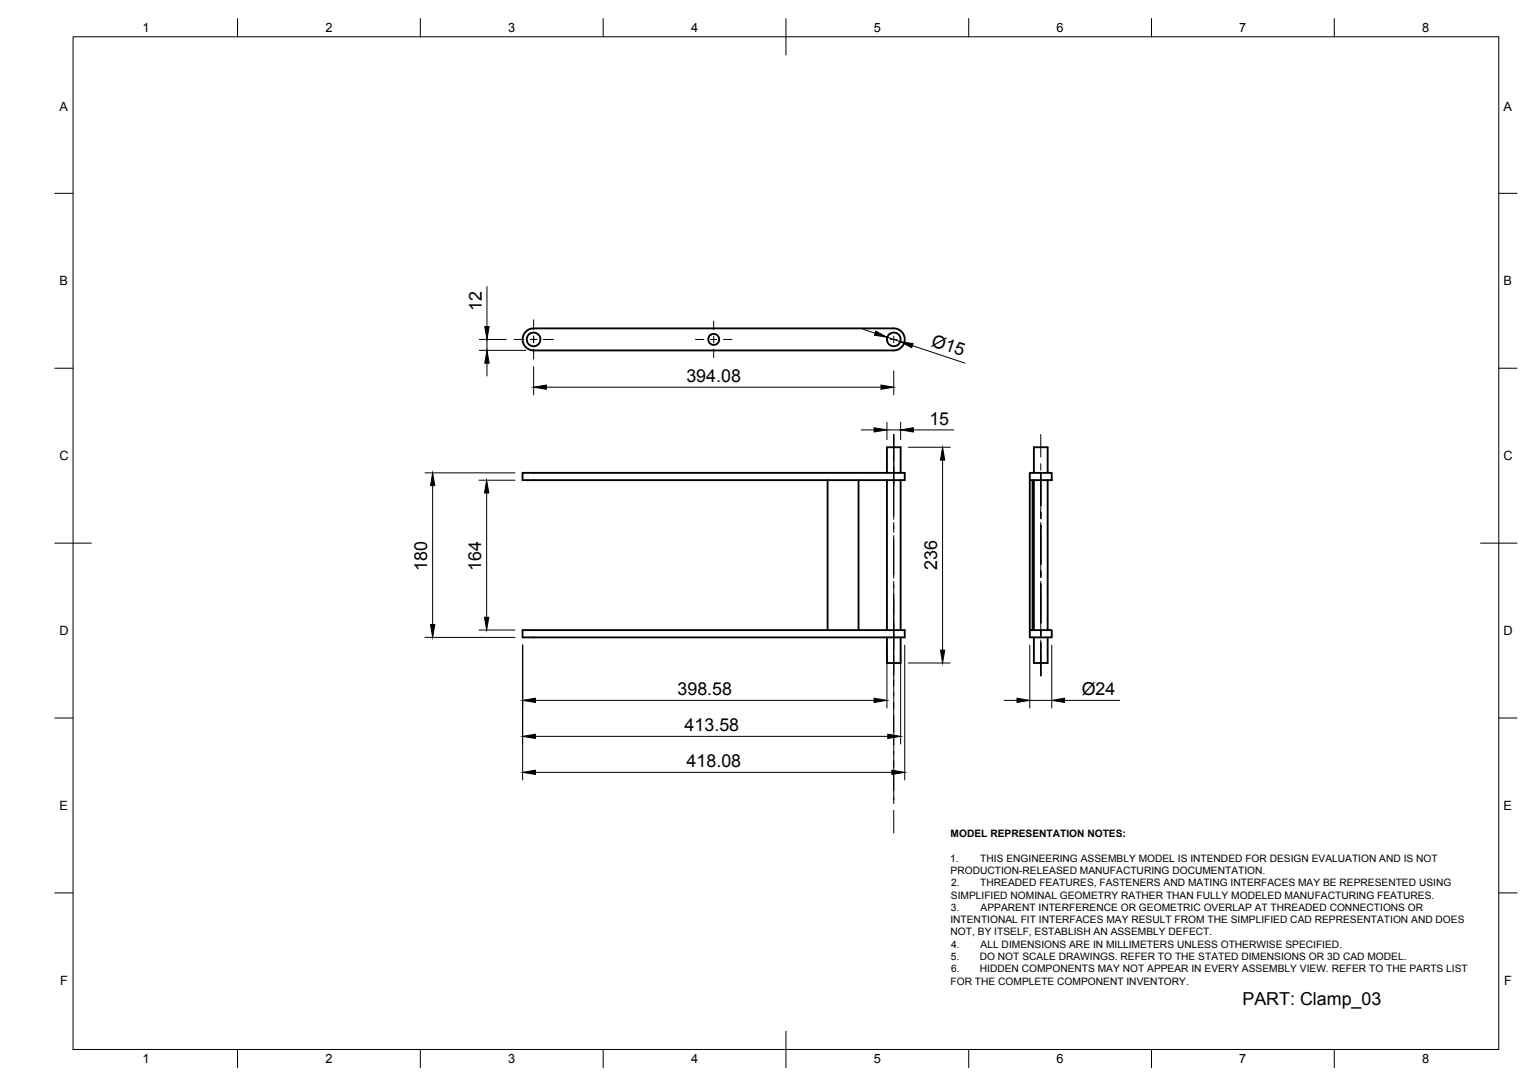
ISO-10303-21;
HEADER;
/* Generated by software containing ST-Developer
 * from STEP Tools, Inc. (www.steptools.com) 
 */

FILE_DESCRIPTION(
/* description */ (''),
/* implementation_level */ '2;1');

FILE_NAME(
/* name */ 'Clamp_03.step',
/* time_stamp */ '2026-10-05T15:35:09-07:00',
/* author */ (''),
/* organization */ (''),
/* preprocessor_version */ 'ST-DEVELOPER v20.2',
/* originating_system */ 'Autodesk Translation Framework v15.15.0.0',
/* authorisation */ '');

FILE_SCHEMA (('AUTOMOTIVE_DESIGN { 1 0 10303 214 3 1 1 }'));
ENDSEC;

DATA;
#10=MECHANICAL_DESIGN_GEOMETRIC_PRESENTATION_REPRESENTATION('',(#544),#74523);
#526=SHAPE_REPRESENTATION_RELATIONSHIP('SRR','None',#74559,#535);
#535=ADVANCED_BREP_SHAPE_REPRESENTATION('',(#553),#74515);
#544=STYLED_ITEM('',(#74612),#553);
#553=MANIFOLD_SOLID_BREP('Body1',#4723);
#569=FACE_BOUND('',#869,.T.);
#570=FACE_BOUND('',#870,.T.);
#571=FACE_BOUND('',#871,.T.);
#572=FACE_BOUND('',#873,.T.);
#573=FACE_BOUND('',#874,.T.);
#574=FACE_BOUND('',#875,.T.);
#575=FACE_BOUND('',#888,.T.);
#576=FACE_BOUND('',#889,.T.);
#577=FACE_BOUND('',#890,.T.);
#578=FACE_BOUND('',#892,.T.);
#579=FACE_BOUND('',#893,.T.);
#580=FACE_BOUND('',#894,.T.);
#623=PLANE('',#4902);
#624=PLANE('',#4906);
#625=PLANE('',#4907);
#626=PLANE('',#4911);
#627=PLANE('',#4912);
#628=PLANE('',#4913);
#629=PLANE('',#4914);
#630=PLANE('',#4915);
#631=PLANE('',#4919);
#632=PLANE('',#4923);
#633=PLANE('',#4927);
#634=PLANE('',#4928);
#708=FACE_OUTER_BOUND('',#860,.T.);
#709=FACE_OUTER_BOUND('',#861,.T.);
#710=FACE_OUTER_BOUND('',#862,.T.);
#711=FACE_OUTER_BOUND('',#863,.T.);
#712=FACE_OUTER_BOUND('',#864,.T.);
#713=FACE_OUTER_BOUND('',#865,.T.);
#714=FACE_OUTER_BOUND('',#866,.T.);
#715=FACE_OUTER_BOUND('',#867,.T.);
#716=FACE_OUTER_BOUND('',#868,.T.);
#717=FACE_OUTER_BOUND('',#872,.T.);
#718=FACE_OUTER_BOUND('',#876,.T.);
#719=FACE_OUTER_BOUND('',#877,.T.);
#720=FACE_OUTER_BOUND('',#878,.T.);
#721=FACE_OUTER_BOUND('',#879,.T.);
#722=FACE_OUTER_BOUND('',#880,.T.);
#723=FACE_OUTER_BOUND('',#881,.T.);
#724=FACE_OUTER_BOUND('',#882,.T.);
#725=FACE_OUTER_BOUND('',#883,.T.);
#726=FACE_OUTER_BOUND('',#884,.T.);
#727=FACE_OUTER_BOUND('',#885,.T.);
#728=FACE_OUTER_BOUND('',#886,.T.);
#729=FACE_OUTER_BOUND('',#887,.T.);
#730=FACE_OUTER_BOUND('',#891,.T.);
#860=EDGE_LOOP('',(#3102,#3103,#3104,#3105));
#861=EDGE_LOOP('',(#3106,#3107,#3108,#3109));
#862=EDGE_LOOP('',(#3110,#3111,#3112,#3113));
#863=EDGE_LOOP('',(#3114,#3115,#3116,#3117));
#864=EDGE_LOOP('',(#3118,#3119,#3120,#3121));
#865=EDGE_LOOP('',(#3122,#3123,#3124,#3125));
#866=EDGE_LOOP('',(#3126,#3127,#3128,#3129));
#867=EDGE_LOOP('',(#3130,#3131,#3132,#3133));
#868=EDGE_LOOP('',(#3134,#3135,#3136,#3137,#3138,#3139,#3140,#3141));
#869=EDGE_LOOP('',(#3142));
#870=EDGE_LOOP('',(#3143));
#871=EDGE_LOOP('',(#3144));
#872=EDGE_LOOP('',(#3145,#3146,#3147,#3148));
#873=EDGE_LOOP('',(#3149));
#874=EDGE_LOOP('',(#3150));
#875=EDGE_LOOP('',(#3151));
#876=EDGE_LOOP('',(#3152,#3153,#3154,#3155));
#877=EDGE_LOOP('',(#3156));
#878=EDGE_LOOP('',(#3157));
#879=EDGE_LOOP('',(#3158,#3159,#3160,#3161));
#880=EDGE_LOOP('',(#3162,#3163,#3164,#3165));
#881=EDGE_LOOP('',(#3166,#3167,#3168,#3169));
#882=EDGE_LOOP('',(#3170,#3171,#3172,#3173));
#883=EDGE_LOOP('',(#3174,#3175,#3176,#3177,#3178,#3179,#3180,#3181,#3182,
#3183,#3184,#3185));
#884=EDGE_LOOP('',(#3186,#3187,#3188,#3189));
#885=EDGE_LOOP('',(#3190,#3191,#3192,#3193));
#886=EDGE_LOOP('',(#3194,#3195,#3196,#3197));
#887=EDGE_LOOP('',(#3198,#3199,#3200,#3201,#3202,#3203,#3204,#3205));
#888=EDGE_LOOP('',(#3206));
#889=EDGE_LOOP('',(#3207));
#890=EDGE_LOOP('',(#3208));
#891=EDGE_LOOP('',(#3209,#3210,#3211,#3212));
#892=EDGE_LOOP('',(#3213));
#893=EDGE_LOOP('',(#3214));
#894=EDGE_LOOP('',(#3215));
#1066=LINE('',#5982,#1263);
#1067=LINE('',#5988,#1264);
#1068=LINE('',#5994,#1265);
#1069=LINE('',#6000,#1266);
#1070=LINE('',#6006,#1267);
#1071=LINE('',#6013,#1268);
#1072=LINE('',#6016,#1269);
#1073=LINE('',#6019,#1270);
#1074=LINE('',#6021,#1271);
#1075=LINE('',#6022,#1272);
#1076=LINE('',#6028,#1273);
#1077=LINE('',#6032,#1274);
#1078=LINE('',#6033,#1275);
#1079=LINE('',#6035,#1276);
#1080=LINE('',#6037,#1277);
#1081=LINE('',#6038,#1278);
#1082=LINE('',#6040,#1279);
#1083=LINE('',#6046,#1280);
#1084=LINE('',#6052,#1281);
#1085=LINE('',#6053,#1282);
#1086=LINE('',#6054,#1283);
#1087=LINE('',#6057,#1284);
#1088=LINE('',#6058,#1285);
#1089=LINE('',#6061,#1286);
#1090=LINE('',#6062,#1287);
#1091=LINE('',#6067,#1288);
#1092=LINE('',#6072,#1289);
#1093=LINE('',#6074,#1290);
#1094=LINE('',#6075,#1291);
#1095=LINE('',#6077,#1292);
#1096=LINE('',#6078,#1293);
#1097=LINE('',#6083,#1294);
#1098=LINE('',#6087,#1295);
#1099=LINE('',#6089,#1296);
#1100=LINE('',#6090,#1297);
#1263=VECTOR('',#5256,6.00000000000001);
#1264=VECTOR('',#5263,6.00000000000001);
#1265=VECTOR('',#5270,7.5);
#1266=VECTOR('',#5277,7.5);
#1267=VECTOR('',#5284,7.5);
#1268=VECTOR('',#5291,10.);
#1269=VECTOR('',#5294,10.);
#1270=VECTOR('',#5297,9.99999999999999);
#1271=VECTOR('',#5298,9.99999999999999);
#1272=VECTOR('',#5299,10.);
#1273=VECTOR('',#5306,10.);
#1274=VECTOR('',#5309,10.);
#1275=VECTOR('',#5310,9.99999999999999);
#1276=VECTOR('',#5311,9.99999999999999);
#1277=VECTOR('',#5312,10.);
#1278=VECTOR('',#5313,9.99999999999999);
#1279=VECTOR('',#5316,9.99999999999999);
#1280=VECTOR('',#5323,7.5);
#1281=VECTOR('',#5330,10.);
#1282=VECTOR('',#5331,10.);
#1283=VECTOR('',#5332,10.);
#1284=VECTOR('',#5335,9.99999999999999);
#1285=VECTOR('',#5336,10.);
#1286=VECTOR('',#5339,10.);
#1287=VECTOR('',#5340,10.);
#1288=VECTOR('',#5345,7.5);
#1289=VECTOR('',#5350,9.99999999999999);
#1290=VECTOR('',#5351,10.);
#1291=VECTOR('',#5352,9.99999999999999);
#1292=VECTOR('',#5353,9.99999999999999);
#1293=VECTOR('',#5354,10.);
#1294=VECTOR('',#5359,10.);
#1295=VECTOR('',#5364,9.99999999999999);
#1296=VECTOR('',#5365,10.);
#1297=VECTOR('',#5366,9.99999999999999);
#1436=CIRCLE('',#4885,6.00000000000001);
#1437=CIRCLE('',#4886,6.00000000000001);
#1438=CIRCLE('',#4888,6.00000000000001);
#1439=CIRCLE('',#4889,6.00000000000001);
#1440=CIRCLE('',#4891,7.5);
#1441=CIRCLE('',#4892,7.5);
#1442=CIRCLE('',#4894,7.5);
#1443=CIRCLE('',#4895,7.5);
#1444=CIRCLE('',#4897,7.5);
#1445=CIRCLE('',#4898,7.5);
#1446=CIRCLE('',#4900,12.);
#1447=CIRCLE('',#4901,12.);
#1448=CIRCLE('',#4904,12.);
#1449=CIRCLE('',#4905,12.);
#1450=CIRCLE('',#4908,7.5);
#1451=CIRCLE('',#4910,7.5);
#1452=CIRCLE('',#4917,7.5);
#1453=CIRCLE('',#4918,7.5);
#1454=CIRCLE('',#4921,12.);
#1455=CIRCLE('',#4922,12.);
#1456=CIRCLE('',#4925,12.);
#1457=CIRCLE('',#4926,12.);
#1570=VERTEX_POINT('',#5979);
#1571=VERTEX_POINT('',#5981);
#1572=VERTEX_POINT('',#5985);
#1573=VERTEX_POINT('',#5987);
#1574=VERTEX_POINT('',#5991);
#1575=VERTEX_POINT('',#5993);
#1576=VERTEX_POINT('',#5997);
#1577=VERTEX_POINT('',#5999);
#1578=VERTEX_POINT('',#6003);
#1579=VERTEX_POINT('',#6005);
#1580=VERTEX_POINT('',#6009);
#1581=VERTEX_POINT('',#6010);
#1582=VERTEX_POINT('',#6012);
#1583=VERTEX_POINT('',#6014);
#1584=VERTEX_POINT('',#6018);
#1585=VERTEX_POINT('',#6020);
#1586=VERTEX_POINT('',#6024);
#1587=VERTEX_POINT('',#6026);
#1588=VERTEX_POINT('',#6030);
#1589=VERTEX_POINT('',#6031);
#1590=VERTEX_POINT('',#6034);
#1591=VERTEX_POINT('',#6036);
#1592=VERTEX_POINT('',#6041);
#1593=VERTEX_POINT('',#6044);
#1594=VERTEX_POINT('',#6050);
#1595=VERTEX_POINT('',#6051);
#1596=VERTEX_POINT('',#6056);
#1597=VERTEX_POINT('',#6060);
#1598=VERTEX_POINT('',#6064);
#1599=VERTEX_POINT('',#6066);
#1600=VERTEX_POINT('',#6070);
#1601=VERTEX_POINT('',#6071);
#1602=VERTEX_POINT('',#6073);
#1603=VERTEX_POINT('',#6076);
#1604=VERTEX_POINT('',#6080);
#1605=VERTEX_POINT('',#6082);
#1606=VERTEX_POINT('',#6086);
#1607=VERTEX_POINT('',#6088);
#2252=EDGE_CURVE('',#1570,#1570,#1436,.T.);
#2253=EDGE_CURVE('',#1570,#1571,#1066,.T.);
#2254=EDGE_CURVE('',#1571,#1571,#1437,.T.);
#2255=EDGE_CURVE('',#1572,#1572,#1438,.T.);
#2256=EDGE_CURVE('',#1572,#1573,#1067,.T.);
#2257=EDGE_CURVE('',#1573,#1573,#1439,.T.);
#2258=EDGE_CURVE('',#1574,#1574,#1440,.T.);
#2259=EDGE_CURVE('',#1574,#1575,#1068,.T.);
#2260=EDGE_CURVE('',#1575,#1575,#1441,.T.);
#2261=EDGE_CURVE('',#1576,#1576,#1442,.T.);
#2262=EDGE_CURVE('',#1576,#1577,#1069,.T.);
#2263=EDGE_CURVE('',#1577,#1577,#1443,.T.);
#2264=EDGE_CURVE('',#1578,#1578,#1444,.T.);
#2265=EDGE_CURVE('',#1578,#1579,#1070,.T.);
#2266=EDGE_CURVE('',#1579,#1579,#1445,.T.);
#2267=EDGE_CURVE('',#1580,#1581,#1446,.T.);
#2268=EDGE_CURVE('',#1581,#1582,#1071,.T.);
#2269=EDGE_CURVE('',#1583,#1582,#1447,.T.);
#2270=EDGE_CURVE('',#1580,#1583,#1072,.T.);
#2271=EDGE_CURVE('',#1584,#1580,#1073,.T.);
#2272=EDGE_CURVE('',#1585,#1583,#1074,.T.);
#2273=EDGE_CURVE('',#1584,#1585,#1075,.T.);
#2274=EDGE_CURVE('',#1586,#1584,#1448,.T.);
#2275=EDGE_CURVE('',#1587,#1585,#1449,.T.);
#2276=EDGE_CURVE('',#1586,#1587,#1076,.T.);
#2277=EDGE_CURVE('',#1588,#1589,#1077,.T.);
#2278=EDGE_CURVE('',#1589,#1587,#1078,.T.);
#2279=EDGE_CURVE('',#1582,#1590,#1079,.T.);
#2280=EDGE_CURVE('',#1590,#1591,#1080,.T.);
#2281=EDGE_CURVE('',#1591,#1588,#1081,.T.);
#2282=EDGE_CURVE('',#1581,#1586,#1082,.T.);
#2283=EDGE_CURVE('',#1592,#1592,#1450,.T.);
#2284=EDGE_CURVE('',#1593,#1593,#1451,.T.);
#2285=EDGE_CURVE('',#1593,#1592,#1083,.T.);
#2286=EDGE_CURVE('',#1594,#1595,#1084,.T.);
#2287=EDGE_CURVE('',#1594,#1589,#1085,.T.);
#2288=EDGE_CURVE('',#1595,#1588,#1086,.T.);
#2289=EDGE_CURVE('',#1595,#1596,#1087,.T.);
#2290=EDGE_CURVE('',#1596,#1591,#1088,.T.);
#2291=EDGE_CURVE('',#1596,#1597,#1089,.T.);
#2292=EDGE_CURVE('',#1597,#1590,#1090,.T.);
#2293=EDGE_CURVE('',#1598,#1598,#1452,.T.);
#2294=EDGE_CURVE('',#1598,#1599,#1091,.T.);
#2295=EDGE_CURVE('',#1599,#1599,#1453,.T.);
#2296=EDGE_CURVE('',#1600,#1601,#1092,.T.);
#2297=EDGE_CURVE('',#1600,#1602,#1093,.T.);
#2298=EDGE_CURVE('',#1602,#1597,#1094,.T.);
#2299=EDGE_CURVE('',#1594,#1603,#1095,.T.);
#2300=EDGE_CURVE('',#1601,#1603,#1096,.T.);
#2301=EDGE_CURVE('',#1604,#1600,#1454,.T.);
#2302=EDGE_CURVE('',#1604,#1605,#1097,.T.);
#2303=EDGE_CURVE('',#1605,#1602,#1455,.T.);
#2304=EDGE_CURVE('',#1606,#1604,#1098,.T.);
#2305=EDGE_CURVE('',#1606,#1607,#1099,.T.);
#2306=EDGE_CURVE('',#1607,#1605,#1100,.T.);
#2307=EDGE_CURVE('',#1601,#1606,#1456,.T.);
#2308=EDGE_CURVE('',#1603,#1607,#1457,.T.);
#3102=ORIENTED_EDGE('',*,*,#2252,.F.);
#3103=ORIENTED_EDGE('',*,*,#2253,.T.);
#3104=ORIENTED_EDGE('',*,*,#2254,.F.);
#3105=ORIENTED_EDGE('',*,*,#2253,.F.);
#3106=ORIENTED_EDGE('',*,*,#2255,.F.);
#3107=ORIENTED_EDGE('',*,*,#2256,.T.);
#3108=ORIENTED_EDGE('',*,*,#2257,.F.);
#3109=ORIENTED_EDGE('',*,*,#2256,.F.);
#3110=ORIENTED_EDGE('',*,*,#2258,.F.);
#3111=ORIENTED_EDGE('',*,*,#2259,.T.);
#3112=ORIENTED_EDGE('',*,*,#2260,.T.);
#3113=ORIENTED_EDGE('',*,*,#2259,.F.);
#3114=ORIENTED_EDGE('',*,*,#2261,.T.);
#3115=ORIENTED_EDGE('',*,*,#2262,.T.);
#3116=ORIENTED_EDGE('',*,*,#2263,.T.);
#3117=ORIENTED_EDGE('',*,*,#2262,.F.);
#3118=ORIENTED_EDGE('',*,*,#2264,.T.);
#3119=ORIENTED_EDGE('',*,*,#2265,.T.);
#3120=ORIENTED_EDGE('',*,*,#2266,.F.);
#3121=ORIENTED_EDGE('',*,*,#2265,.F.);
#3122=ORIENTED_EDGE('',*,*,#2267,.T.);
#3123=ORIENTED_EDGE('',*,*,#2268,.T.);
#3124=ORIENTED_EDGE('',*,*,#2269,.F.);
#3125=ORIENTED_EDGE('',*,*,#2270,.F.);
#3126=ORIENTED_EDGE('',*,*,#2271,.T.);
#3127=ORIENTED_EDGE('',*,*,#2270,.T.);
#3128=ORIENTED_EDGE('',*,*,#2272,.F.);
#3129=ORIENTED_EDGE('',*,*,#2273,.F.);
#3130=ORIENTED_EDGE('',*,*,#2274,.T.);
#3131=ORIENTED_EDGE('',*,*,#2273,.T.);
#3132=ORIENTED_EDGE('',*,*,#2275,.F.);
#3133=ORIENTED_EDGE('',*,*,#2276,.F.);
#3134=ORIENTED_EDGE('',*,*,#2277,.T.);
#3135=ORIENTED_EDGE('',*,*,#2278,.T.);
#3136=ORIENTED_EDGE('',*,*,#2275,.T.);
#3137=ORIENTED_EDGE('',*,*,#2272,.T.);
#3138=ORIENTED_EDGE('',*,*,#2269,.T.);
#3139=ORIENTED_EDGE('',*,*,#2279,.T.);
#3140=ORIENTED_EDGE('',*,*,#2280,.T.);
#3141=ORIENTED_EDGE('',*,*,#2281,.T.);
#3142=ORIENTED_EDGE('',*,*,#2252,.T.);
#3143=ORIENTED_EDGE('',*,*,#2261,.F.);
#3144=ORIENTED_EDGE('',*,*,#2266,.T.);
#3145=ORIENTED_EDGE('',*,*,#2274,.F.);
#3146=ORIENTED_EDGE('',*,*,#2282,.F.);
#3147=ORIENTED_EDGE('',*,*,#2267,.F.);
#3148=ORIENTED_EDGE('',*,*,#2271,.F.);
#3149=ORIENTED_EDGE('',*,*,#2254,.T.);
#3150=ORIENTED_EDGE('',*,*,#2283,.F.);
#3151=ORIENTED_EDGE('',*,*,#2264,.F.);
#3152=ORIENTED_EDGE('',*,*,#2284,.T.);
#3153=ORIENTED_EDGE('',*,*,#2285,.T.);
#3154=ORIENTED_EDGE('',*,*,#2283,.T.);
#3155=ORIENTED_EDGE('',*,*,#2285,.F.);
#3156=ORIENTED_EDGE('',*,*,#2284,.F.);
#3157=ORIENTED_EDGE('',*,*,#2260,.F.);
#3158=ORIENTED_EDGE('',*,*,#2286,.F.);
#3159=ORIENTED_EDGE('',*,*,#2287,.T.);
#3160=ORIENTED_EDGE('',*,*,#2277,.F.);
#3161=ORIENTED_EDGE('',*,*,#2288,.F.);
#3162=ORIENTED_EDGE('',*,*,#2289,.F.);
#3163=ORIENTED_EDGE('',*,*,#2288,.T.);
#3164=ORIENTED_EDGE('',*,*,#2281,.F.);
#3165=ORIENTED_EDGE('',*,*,#2290,.F.);
#3166=ORIENTED_EDGE('',*,*,#2291,.F.);
#3167=ORIENTED_EDGE('',*,*,#2290,.T.);
#3168=ORIENTED_EDGE('',*,*,#2280,.F.);
#3169=ORIENTED_EDGE('',*,*,#2292,.F.);
#3170=ORIENTED_EDGE('',*,*,#2293,.T.);
#3171=ORIENTED_EDGE('',*,*,#2294,.T.);
#3172=ORIENTED_EDGE('',*,*,#2295,.F.);
#3173=ORIENTED_EDGE('',*,*,#2294,.F.);
#3174=ORIENTED_EDGE('',*,*,#2296,.F.);
#3175=ORIENTED_EDGE('',*,*,#2297,.T.);
#3176=ORIENTED_EDGE('',*,*,#2298,.T.);
#3177=ORIENTED_EDGE('',*,*,#2292,.T.);
#3178=ORIENTED_EDGE('',*,*,#2279,.F.);
#3179=ORIENTED_EDGE('',*,*,#2268,.F.);
#3180=ORIENTED_EDGE('',*,*,#2282,.T.);
#3181=ORIENTED_EDGE('',*,*,#2276,.T.);
#3182=ORIENTED_EDGE('',*,*,#2278,.F.);
#3183=ORIENTED_EDGE('',*,*,#2287,.F.);
#3184=ORIENTED_EDGE('',*,*,#2299,.T.);
#3185=ORIENTED_EDGE('',*,*,#2300,.F.);
#3186=ORIENTED_EDGE('',*,*,#2301,.F.);
#3187=ORIENTED_EDGE('',*,*,#2302,.T.);
#3188=ORIENTED_EDGE('',*,*,#2303,.T.);
#3189=ORIENTED_EDGE('',*,*,#2297,.F.);
#3190=ORIENTED_EDGE('',*,*,#2304,.F.);
#3191=ORIENTED_EDGE('',*,*,#2305,.T.);
#3192=ORIENTED_EDGE('',*,*,#2306,.T.);
#3193=ORIENTED_EDGE('',*,*,#2302,.F.);
#3194=ORIENTED_EDGE('',*,*,#2307,.F.);
#3195=ORIENTED_EDGE('',*,*,#2300,.T.);
#3196=ORIENTED_EDGE('',*,*,#2308,.T.);
#3197=ORIENTED_EDGE('',*,*,#2305,.F.);
#3198=ORIENTED_EDGE('',*,*,#2291,.T.);
#3199=ORIENTED_EDGE('',*,*,#2298,.F.);
#3200=ORIENTED_EDGE('',*,*,#2303,.F.);
#3201=ORIENTED_EDGE('',*,*,#2306,.F.);
#3202=ORIENTED_EDGE('',*,*,#2308,.F.);
#3203=ORIENTED_EDGE('',*,*,#2299,.F.);
#3204=ORIENTED_EDGE('',*,*,#2286,.T.);
#3205=ORIENTED_EDGE('',*,*,#2289,.T.);
#3206=ORIENTED_EDGE('',*,*,#2255,.T.);
#3207=ORIENTED_EDGE('',*,*,#2263,.F.);
#3208=ORIENTED_EDGE('',*,*,#2293,.F.);
#3209=ORIENTED_EDGE('',*,*,#2307,.T.);
#3210=ORIENTED_EDGE('',*,*,#2304,.T.);
#3211=ORIENTED_EDGE('',*,*,#2301,.T.);
#3212=ORIENTED_EDGE('',*,*,#2296,.T.);
#3213=ORIENTED_EDGE('',*,*,#2257,.T.);
#3214=ORIENTED_EDGE('',*,*,#2258,.T.);
#3215=ORIENTED_EDGE('',*,*,#2295,.T.);
#4526=CYLINDRICAL_SURFACE('',#4884,6.00000000000001);
#4527=CYLINDRICAL_SURFACE('',#4887,6.00000000000001);
#4528=CYLINDRICAL_SURFACE('',#4890,7.5);
#4529=CYLINDRICAL_SURFACE('',#4893,7.5);
#4530=CYLINDRICAL_SURFACE('',#4896,7.5);
#4531=CYLINDRICAL_SURFACE('',#4899,12.);
#4532=CYLINDRICAL_SURFACE('',#4903,12.);
#4533=CYLINDRICAL_SURFACE('',#4909,7.5);
#4534=CYLINDRICAL_SURFACE('',#4916,7.5);
#4535=CYLINDRICAL_SURFACE('',#4920,12.);
#4536=CYLINDRICAL_SURFACE('',#4924,12.);
#4604=ADVANCED_FACE('',(#708),#4526,.F.);
#4605=ADVANCED_FACE('',(#709),#4527,.F.);
#4606=ADVANCED_FACE('',(#710),#4528,.T.);
#4607=ADVANCED_FACE('',(#711),#4529,.T.);
#4608=ADVANCED_FACE('',(#712),#4530,.F.);
#4609=ADVANCED_FACE('',(#713),#4531,.T.);
#4610=ADVANCED_FACE('',(#714),#623,.T.);
#4611=ADVANCED_FACE('',(#715),#4532,.T.);
#4612=ADVANCED_FACE('',(#716,#569,#570,#571),#624,.T.);
#4613=ADVANCED_FACE('',(#717,#572,#573,#574),#625,.F.);
#4614=ADVANCED_FACE('',(#718),#4533,.T.);
#4615=ADVANCED_FACE('',(#719),#626,.T.);
#4616=ADVANCED_FACE('',(#720),#627,.F.);
#4617=ADVANCED_FACE('',(#721),#628,.T.);
#4618=ADVANCED_FACE('',(#722),#629,.T.);
#4619=ADVANCED_FACE('',(#723),#630,.T.);
#4620=ADVANCED_FACE('',(#724),#4534,.F.);
#4621=ADVANCED_FACE('',(#725),#631,.F.);
#4622=ADVANCED_FACE('',(#726),#4535,.T.);
#4623=ADVANCED_FACE('',(#727),#632,.F.);
#4624=ADVANCED_FACE('',(#728),#4536,.T.);
#4625=ADVANCED_FACE('',(#729,#575,#576,#577),#633,.F.);
#4626=ADVANCED_FACE('',(#730,#578,#579,#580),#634,.T.);
#4723=CLOSED_SHELL('',(#4604,#4605,#4606,#4607,#4608,#4609,#4610,#4611,
#4612,#4613,#4614,#4615,#4616,#4617,#4618,#4619,#4620,#4621,#4622,#4623,
#4624,#4625,#4626));
#4883=AXIS2_PLACEMENT_3D('',#5977,#5250,#5251);
#4884=AXIS2_PLACEMENT_3D('',#5978,#5252,#5253);
#4885=AXIS2_PLACEMENT_3D('',#5980,#5254,#5255);
#4886=AXIS2_PLACEMENT_3D('',#5983,#5257,#5258);
#4887=AXIS2_PLACEMENT_3D('',#5984,#5259,#5260);
#4888=AXIS2_PLACEMENT_3D('',#5986,#5261,#5262);
#4889=AXIS2_PLACEMENT_3D('',#5989,#5264,#5265);
#4890=AXIS2_PLACEMENT_3D('',#5990,#5266,#5267);
#4891=AXIS2_PLACEMENT_3D('',#5992,#5268,#5269);
#4892=AXIS2_PLACEMENT_3D('',#5995,#5271,#5272);
#4893=AXIS2_PLACEMENT_3D('',#5996,#5273,#5274);
#4894=AXIS2_PLACEMENT_3D('',#5998,#5275,#5276);
#4895=AXIS2_PLACEMENT_3D('',#6001,#5278,#5279);
#4896=AXIS2_PLACEMENT_3D('',#6002,#5280,#5281);
#4897=AXIS2_PLACEMENT_3D('',#6004,#5282,#5283);
#4898=AXIS2_PLACEMENT_3D('',#6007,#5285,#5286);
#4899=AXIS2_PLACEMENT_3D('',#6008,#5287,#5288);
#4900=AXIS2_PLACEMENT_3D('',#6011,#5289,#5290);
#4901=AXIS2_PLACEMENT_3D('',#6015,#5292,#5293);
#4902=AXIS2_PLACEMENT_3D('',#6017,#5295,#5296);
#4903=AXIS2_PLACEMENT_3D('',#6023,#5300,#5301);
#4904=AXIS2_PLACEMENT_3D('',#6025,#5302,#5303);
#4905=AXIS2_PLACEMENT_3D('',#6027,#5304,#5305);
#4906=AXIS2_PLACEMENT_3D('',#6029,#5307,#5308);
#4907=AXIS2_PLACEMENT_3D('',#6039,#5314,#5315);
#4908=AXIS2_PLACEMENT_3D('',#6042,#5317,#5318);
#4909=AXIS2_PLACEMENT_3D('',#6043,#5319,#5320);
#4910=AXIS2_PLACEMENT_3D('',#6045,#5321,#5322);
#4911=AXIS2_PLACEMENT_3D('',#6047,#5324,#5325);
#4912=AXIS2_PLACEMENT_3D('',#6048,#5326,#5327);
#4913=AXIS2_PLACEMENT_3D('',#6049,#5328,#5329);
#4914=AXIS2_PLACEMENT_3D('',#6055,#5333,#5334);
#4915=AXIS2_PLACEMENT_3D('',#6059,#5337,#5338);
#4916=AXIS2_PLACEMENT_3D('',#6063,#5341,#5342);
#4917=AXIS2_PLACEMENT_3D('',#6065,#5343,#5344);
#4918=AXIS2_PLACEMENT_3D('',#6068,#5346,#5347);
#4919=AXIS2_PLACEMENT_3D('',#6069,#5348,#5349);
#4920=AXIS2_PLACEMENT_3D('',#6079,#5355,#5356);
#4921=AXIS2_PLACEMENT_3D('',#6081,#5357,#5358);
#4922=AXIS2_PLACEMENT_3D('',#6084,#5360,#5361);
#4923=AXIS2_PLACEMENT_3D('',#6085,#5362,#5363);
#4924=AXIS2_PLACEMENT_3D('',#6091,#5367,#5368);
#4925=AXIS2_PLACEMENT_3D('',#6092,#5369,#5370);
#4926=AXIS2_PLACEMENT_3D('',#6093,#5371,#5372);
#4927=AXIS2_PLACEMENT_3D('',#6094,#5373,#5374);
#4928=AXIS2_PLACEMENT_3D('',#6095,#5375,#5376);
#5250=DIRECTION('axis',(0.,0.,1.));
#5251=DIRECTION('refdir',(1.,0.,0.));
#5252=DIRECTION('center_axis',(0.,-1.,0.));
#5253=DIRECTION('ref_axis',(1.,0.,0.));
#5254=DIRECTION('center_axis',(0.,-1.,0.));
#5255=DIRECTION('ref_axis',(1.,0.,0.));
#5256=DIRECTION('',(0.,-1.,0.));
#5257=DIRECTION('center_axis',(0.,1.,0.));
#5258=DIRECTION('ref_axis',(1.,0.,0.));
#5259=DIRECTION('center_axis',(0.,1.,0.));
#5260=DIRECTION('ref_axis',(1.,0.,0.));
#5261=DIRECTION('center_axis',(0.,1.,0.));
#5262=DIRECTION('ref_axis',(1.,0.,0.));
#5263=DIRECTION('',(0.,1.,0.));
#5264=DIRECTION('center_axis',(0.,-1.,0.));
#5265=DIRECTION('ref_axis',(1.,0.,0.));
#5266=DIRECTION('center_axis',(-3.66477378287572E-33,-1.,2.99251489117293E-17));
#5267=DIRECTION('ref_axis',(1.,3.66477378287573E-33,2.44929359829471E-16));
#5268=DIRECTION('center_axis',(0.,-1.,0.));
#5269=DIRECTION('ref_axis',(1.,0.,0.));
#5270=DIRECTION('',(3.66477378287572E-33,1.,-2.99251489117293E-17));
#5271=DIRECTION('center_axis',(-3.66477378287572E-33,-1.,2.99251489117293E-17));
#5272=DIRECTION('ref_axis',(1.,3.66477378287573E-33,2.44929359829471E-16));
#5273=DIRECTION('center_axis',(-3.66477378287572E-33,-1.,2.99251489117293E-17));
#5274=DIRECTION('ref_axis',(1.,3.66477378287573E-33,2.44929359829471E-16));
#5275=DIRECTION('center_axis',(0.,1.,0.));
#5276=DIRECTION('ref_axis',(1.,0.,2.44929359829471E-16));
#5277=DIRECTION('',(3.66477378287572E-33,1.,-2.99251489117293E-17));
#5278=DIRECTION('center_axis',(0.,-1.,0.));
#5279=DIRECTION('ref_axis',(1.,0.,0.));
#5280=DIRECTION('center_axis',(0.,1.,0.));
#5281=DIRECTION('ref_axis',(1.,0.,0.));
#5282=DIRECTION('center_axis',(0.,-1.,0.));
#5283=DIRECTION('ref_axis',(1.,0.,0.));
#5284=DIRECTION('',(0.,1.,0.));
#5285=DIRECTION('center_axis',(0.,-1.,0.));
#5286=DIRECTION('ref_axis',(1.,0.,0.));
#5287=DIRECTION('center_axis',(0.,1.,0.));
#5288=DIRECTION('ref_axis',(0.812015371342714,0.,0.583636048152574));
#5289=DIRECTION('center_axis',(0.,1.,0.));
#5290=DIRECTION('ref_axis',(0.812015371342714,0.,0.583636048152574));
#5291=DIRECTION('',(0.,1.,0.));
#5292=DIRECTION('center_axis',(0.,1.,0.));
#5293=DIRECTION('ref_axis',(0.812015371342714,0.,0.583636048152574));
#5294=DIRECTION('',(0.,1.,0.));
#5295=DIRECTION('center_axis',(0.812015371342714,0.,0.583636048152575));
#5296=DIRECTION('ref_axis',(0.583636048152575,0.,-0.812015371342714));
#5297=DIRECTION('',(0.583636048152575,0.,-0.812015371342714));
#5298=DIRECTION('',(0.583636048152575,0.,-0.812015371342714));
#5299=DIRECTION('',(0.,1.,0.));
#5300=DIRECTION('center_axis',(0.,1.,0.));
#5301=DIRECTION('ref_axis',(-0.812015371342714,0.,-0.583636048152575));
#5302=DIRECTION('center_axis',(0.,1.,0.));
#5303=DIRECTION('ref_axis',(-0.812015371342714,0.,-0.583636048152575));
#5304=DIRECTION('center_axis',(0.,1.,0.));
#5305=DIRECTION('ref_axis',(-0.812015371342714,0.,-0.583636048152575));
#5306=DIRECTION('',(0.,1.,0.));
#5307=DIRECTION('center_axis',(0.,1.,0.));
#5308=DIRECTION('ref_axis',(1.,0.,0.));
#5309=DIRECTION('',(-0.812015371342711,0.,-0.583636048152579));
#5310=DIRECTION('',(-0.583636048152575,0.,0.812015371342714));
#5311=DIRECTION('',(-0.583636048152575,0.,0.812015371342714));
#5312=DIRECTION('',(0.812015371342709,0.,0.583636048152581));
#5313=DIRECTION('',(-0.583636048152575,0.,0.812015371342714));
#5314=DIRECTION('center_axis',(0.,1.,0.));
#5315=DIRECTION('ref_axis',(1.,0.,0.));
#5316=DIRECTION('',(-0.583636048152575,0.,0.812015371342714));
#5317=DIRECTION('center_axis',(0.,-1.,0.));
#5318=DIRECTION('ref_axis',(1.,0.,2.44929359829471E-16));
#5319=DIRECTION('center_axis',(-3.66477378287572E-33,-1.,2.99251489117293E-17));
#5320=DIRECTION('ref_axis',(1.,3.66477378287573E-33,2.44929359829471E-16));
#5321=DIRECTION('center_axis',(3.66477378287572E-33,1.,-2.99251489117293E-17));
#5322=DIRECTION('ref_axis',(1.,3.66477378287573E-33,2.44929359829471E-16));
#5323=DIRECTION('',(3.66477378287572E-33,1.,-2.99251489117293E-17));
#5324=DIRECTION('center_axis',(-3.66477378287572E-33,-1.,2.99251489117293E-17));
#5325=DIRECTION('ref_axis',(1.,3.66477378287573E-33,2.44929359829471E-16));
#5326=DIRECTION('center_axis',(-3.66477378287572E-33,-1.,2.99251489117293E-17));
#5327=DIRECTION('ref_axis',(1.,3.66477378287573E-33,2.44929359829471E-16));
#5328=DIRECTION('center_axis',(-0.583636048152579,0.,0.812015371342711));
#5329=DIRECTION('ref_axis',(-0.812015371342711,0.,-0.583636048152579));
#5330=DIRECTION('',(0.812015371342711,0.,0.583636048152579));
#5331=DIRECTION('',(0.,-1.,0.));
#5332=DIRECTION('',(0.,-1.,0.));
#5333=DIRECTION('center_axis',(0.812015371342714,0.,0.583636048152575));
#5334=DIRECTION('ref_axis',(-0.583636048152575,0.,0.812015371342714));
#5335=DIRECTION('',(0.583636048152575,0.,-0.812015371342714));
#5336=DIRECTION('',(0.,-1.,0.));
#5337=DIRECTION('center_axis',(0.583636048152581,0.,-0.812015371342709));
#5338=DIRECTION('ref_axis',(0.812015371342709,0.,0.583636048152581));
#5339=DIRECTION('',(-0.812015371342709,0.,-0.583636048152581));
#5340=DIRECTION('',(0.,-1.,0.));
#5341=DIRECTION('center_axis',(0.,1.,0.));
#5342=DIRECTION('ref_axis',(1.,0.,0.));
#5343=DIRECTION('center_axis',(0.,-1.,0.));
#5344=DIRECTION('ref_axis',(1.,0.,0.));
#5345=DIRECTION('',(0.,1.,0.));
#5346=DIRECTION('center_axis',(0.,-1.,0.));
#5347=DIRECTION('ref_axis',(1.,0.,0.));
#5348=DIRECTION('center_axis',(0.812015371342714,0.,0.583636048152575));
#5349=DIRECTION('ref_axis',(-0.583636048152575,0.,0.812015371342714));
#5350=DIRECTION('',(-0.583636048152575,0.,0.812015371342714));
#5351=DIRECTION('',(0.,-1.,0.));
#5352=DIRECTION('',(-0.583636048152575,0.,0.812015371342714));
#5353=DIRECTION('',(-0.583636048152575,0.,0.812015371342714));
#5354=DIRECTION('',(0.,-1.,0.));
#5355=DIRECTION('center_axis',(0.,1.,0.));
#5356=DIRECTION('ref_axis',(0.812015371342714,0.,0.583636048152574));
#5357=DIRECTION('center_axis',(0.,1.,0.));
#5358=DIRECTION('ref_axis',(0.812015371342714,0.,0.583636048152574));
#5359=DIRECTION('',(0.,-1.,0.));
#5360=DIRECTION('center_axis',(0.,1.,0.));
#5361=DIRECTION('ref_axis',(0.812015371342714,0.,0.583636048152574));
#5362=DIRECTION('center_axis',(-0.812015371342714,0.,-0.583636048152575));
#5363=DIRECTION('ref_axis',(0.583636048152575,0.,-0.812015371342714));
#5364=DIRECTION('',(0.583636048152575,0.,-0.812015371342714));
#5365=DIRECTION('',(0.,-1.,0.));
#5366=DIRECTION('',(0.583636048152575,0.,-0.812015371342714));
#5367=DIRECTION('center_axis',(0.,1.,0.));
#5368=DIRECTION('ref_axis',(-0.812015371342714,0.,-0.583636048152575));
#5369=DIRECTION('center_axis',(0.,1.,0.));
#5370=DIRECTION('ref_axis',(-0.812015371342714,0.,-0.583636048152575));
#5371=DIRECTION('center_axis',(0.,1.,0.));
#5372=DIRECTION('ref_axis',(-0.812015371342714,0.,-0.583636048152575));
#5373=DIRECTION('center_axis',(0.,1.,0.));
#5374=DIRECTION('ref_axis',(1.,0.,0.));
#5375=DIRECTION('center_axis',(0.,1.,0.));
#5376=DIRECTION('ref_axis',(1.,0.,0.));
#5977=CARTESIAN_POINT('',(0.,0.,0.));
#5978=CARTESIAN_POINT('Origin',(60.231676812499,-90.,175.));
#5979=CARTESIAN_POINT('',(54.231676812499,-82.,175.));
#5980=CARTESIAN_POINT('Origin',(60.231676812499,-82.,175.));
#5981=CARTESIAN_POINT('',(54.231676812499,-90.,175.));
#5982=CARTESIAN_POINT('',(54.231676812499,-90.,175.));
#5983=CARTESIAN_POINT('Origin',(60.231676812499,-90.,175.));
#5984=CARTESIAN_POINT('Origin',(60.231676812499,-90.,175.));
#5985=CARTESIAN_POINT('',(54.231676812499,82.,175.));
#5986=CARTESIAN_POINT('Origin',(60.231676812499,82.,175.));
#5987=CARTESIAN_POINT('',(54.231676812499,90.,175.));
#5988=CARTESIAN_POINT('',(54.231676812499,-90.,175.));
#5989=CARTESIAN_POINT('Origin',(60.231676812499,90.,175.));
#5990=CARTESIAN_POINT('Origin',(-54.768323187501,4.78802382587669E-15,335.));
#5991=CARTESIAN_POINT('',(-62.268323187501,90.,335.));
#5992=CARTESIAN_POINT('Origin',(-54.768323187501,90.,335.));
#5993=CARTESIAN_POINT('',(-62.268323187501,118.,335.));
#5994=CARTESIAN_POINT('',(-62.268323187501,4.78802382587669E-15,335.));
#5995=CARTESIAN_POINT('Origin',(-54.768323187501,118.,335.));
#5996=CARTESIAN_POINT('Origin',(-54.768323187501,4.78802382587669E-15,335.));
#5997=CARTESIAN_POINT('',(-62.268323187501,-82.,335.));
#5998=CARTESIAN_POINT('Origin',(-54.768323187501,-82.,335.));
#5999=CARTESIAN_POINT('',(-62.268323187501,82.,335.));
#6000=CARTESIAN_POINT('',(-62.268323187501,4.78802382587669E-15,335.));
#6001=CARTESIAN_POINT('Origin',(-54.768323187501,82.,335.));
#6002=CARTESIAN_POINT('Origin',(175.231676812499,-90.,15.));
#6003=CARTESIAN_POINT('',(167.731676812499,-90.,15.));
#6004=CARTESIAN_POINT('Origin',(175.231676812499,-90.,15.));
#6005=CARTESIAN_POINT('',(167.731676812499,-82.,15.));
#6006=CARTESIAN_POINT('',(167.731676812499,-90.,15.));
#6007=CARTESIAN_POINT('Origin',(175.231676812499,-82.,15.));
#6008=CARTESIAN_POINT('Origin',(175.231676812499,-90.,15.));
#6009=CARTESIAN_POINT('',(184.975861268612,-90.,22.0036325778309));
#6010=CARTESIAN_POINT('',(165.487492356386,-90.,7.99636742216909));
#6011=CARTESIAN_POINT('Origin',(175.231676812499,-90.,15.));
#6012=CARTESIAN_POINT('',(165.487492356386,-82.,7.99636742216912));
#6013=CARTESIAN_POINT('',(165.487492356386,-90.,7.99636742216909));
#6014=CARTESIAN_POINT('',(184.975861268612,-82.,22.0036325778309));
#6015=CARTESIAN_POINT('Origin',(175.231676812499,-82.,15.));
#6016=CARTESIAN_POINT('',(184.975861268612,-90.,22.0036325778309));
#6017=CARTESIAN_POINT('Origin',(-45.0241387313884,-90.,342.003632577831));
#6018=CARTESIAN_POINT('',(-45.0241387313884,-90.,342.003632577831));
#6019=CARTESIAN_POINT('',(-45.0241387313884,-90.,342.003632577831));
#6020=CARTESIAN_POINT('',(-45.0241387313884,-82.,342.003632577831));
#6021=CARTESIAN_POINT('',(-45.0241387313884,-82.,342.003632577831));
#6022=CARTESIAN_POINT('',(-45.0241387313884,-90.,342.003632577831));
#6023=CARTESIAN_POINT('Origin',(-54.768323187501,-90.,335.));
#6024=CARTESIAN_POINT('',(-64.5125076436135,-90.,327.996367422169));
#6025=CARTESIAN_POINT('Origin',(-54.768323187501,-90.,335.));
#6026=CARTESIAN_POINT('',(-64.5125076436135,-82.,327.996367422169));
#6027=CARTESIAN_POINT('Origin',(-54.768323187501,-82.,335.));
#6028=CARTESIAN_POINT('',(-64.5125076436135,-90.,327.996367422169));
#6029=CARTESIAN_POINT('Origin',(60.231676812499,-82.,175.));
#6030=CARTESIAN_POINT('',(-39.60939337502,-82.,298.488745960275));
#6031=CARTESIAN_POINT('',(-42.0454394890482,-82.,296.737837815817));
#6032=CARTESIAN_POINT('',(-42.0454394890482,-82.,296.737837815817));
#6033=CARTESIAN_POINT('',(165.487492356386,-82.,7.99636742216909));
#6034=CARTESIAN_POINT('',(-22.280326233118,-82.,269.238549807567));
#6035=CARTESIAN_POINT('',(165.487492356386,-82.,7.99636742216909));
#6036=CARTESIAN_POINT('',(-19.8442801190899,-82.,270.989457952024));
#6037=CARTESIAN_POINT('',(-22.280326233118,-82.,269.238549807567));
#6038=CARTESIAN_POINT('',(167.923538470415,-82.,9.74727556662682));
#6039=CARTESIAN_POINT('Origin',(60.231676812499,-90.,175.));
#6040=CARTESIAN_POINT('',(165.487492356386,-90.,7.99636742216909));
#6041=CARTESIAN_POINT('',(-62.268323187501,-90.,335.));
#6042=CARTESIAN_POINT('Origin',(-54.768323187501,-90.,335.));
#6043=CARTESIAN_POINT('Origin',(-54.768323187501,4.78802382587669E-15,335.));
#6044=CARTESIAN_POINT('',(-62.268323187501,-118.,335.));
#6045=CARTESIAN_POINT('Origin',(-54.768323187501,-118.,335.));
#6046=CARTESIAN_POINT('',(-62.268323187501,4.78802382587669E-15,335.));
#6047=CARTESIAN_POINT('Origin',(-54.768323187501,-118.,335.));
#6048=CARTESIAN_POINT('Origin',(-54.768323187501,118.,335.));
#6049=CARTESIAN_POINT('Origin',(-39.60939337502,82.,298.488745960275));
#6050=CARTESIAN_POINT('',(-42.0454394890482,82.,296.737837815817));
#6051=CARTESIAN_POINT('',(-39.60939337502,82.,298.488745960275));
#6052=CARTESIAN_POINT('',(-35.9553242039781,82.,301.115108176961));
#6053=CARTESIAN_POINT('',(-42.0454394890482,82.,296.737837815817));
#6054=CARTESIAN_POINT('',(-39.60939337502,82.,298.488745960275));
#6055=CARTESIAN_POINT('Origin',(-19.84428011909,82.,270.989457952024));
#6056=CARTESIAN_POINT('',(-19.8442801190899,82.,270.989457952024));
#6057=CARTESIAN_POINT('',(16.5396291756623,82.,220.368366759326));
#6058=CARTESIAN_POINT('',(-19.8442801190899,82.,270.989457952024));
#6059=CARTESIAN_POINT('Origin',(-22.280326233118,82.,269.238549807567));
#6060=CARTESIAN_POINT('',(-22.280326233118,82.,269.238549807567));
#6061=CARTESIAN_POINT('',(-17.4082340050621,82.,272.740366096482));
#6062=CARTESIAN_POINT('',(-22.280326233118,82.,269.238549807567));
#6063=CARTESIAN_POINT('Origin',(175.231676812499,90.,15.));
#6064=CARTESIAN_POINT('',(167.731676812499,82.,15.));
#6065=CARTESIAN_POINT('Origin',(175.231676812499,82.,15.));
#6066=CARTESIAN_POINT('',(167.731676812499,90.,15.));
#6067=CARTESIAN_POINT('',(167.731676812499,90.,15.));
#6068=CARTESIAN_POINT('Origin',(175.231676812499,90.,15.));
#6069=CARTESIAN_POINT('Origin',(165.487492356386,90.,7.99636742216909));
#6070=CARTESIAN_POINT('',(165.487492356386,90.,7.99636742216909));
#6071=CARTESIAN_POINT('',(-64.5125076436135,90.,327.996367422169));
#6072=CARTESIAN_POINT('',(165.487492356386,90.,7.99636742216909));
#6073=CARTESIAN_POINT('',(165.487492356386,82.,7.99636742216912));
#6074=CARTESIAN_POINT('',(165.487492356386,90.,7.99636742216909));
#6075=CARTESIAN_POINT('',(165.487492356386,82.,7.99636742216909));
#6076=CARTESIAN_POINT('',(-64.5125076436135,82.,327.996367422169));
#6077=CARTESIAN_POINT('',(165.487492356386,82.,7.99636742216909));
#6078=CARTESIAN_POINT('',(-64.5125076436135,90.,327.996367422169));
#6079=CARTESIAN_POINT('Origin',(175.231676812499,90.,15.));
#6080=CARTESIAN_POINT('',(184.975861268612,90.,22.0036325778309));
#6081=CARTESIAN_POINT('Origin',(175.231676812499,90.,15.));
#6082=CARTESIAN_POINT('',(184.975861268612,82.,22.0036325778309));
#6083=CARTESIAN_POINT('',(184.975861268612,90.,22.0036325778309));
#6084=CARTESIAN_POINT('Origin',(175.231676812499,82.,15.));
#6085=CARTESIAN_POINT('Origin',(-45.0241387313884,90.,342.003632577831));
#6086=CARTESIAN_POINT('',(-45.0241387313884,90.,342.003632577831));
#6087=CARTESIAN_POINT('',(-45.0241387313884,90.,342.003632577831));
#6088=CARTESIAN_POINT('',(-45.0241387313884,82.,342.003632577831));
#6089=CARTESIAN_POINT('',(-45.0241387313884,90.,342.003632577831));
#6090=CARTESIAN_POINT('',(-45.0241387313884,82.,342.003632577831));
#6091=CARTESIAN_POINT('Origin',(-54.768323187501,90.,335.));
#6092=CARTESIAN_POINT('Origin',(-54.768323187501,90.,335.));
#6093=CARTESIAN_POINT('Origin',(-54.768323187501,82.,335.));
#6094=CARTESIAN_POINT('Origin',(60.231676812499,82.,175.));
#6095=CARTESIAN_POINT('Origin',(60.231676812499,90.,175.));
#74504=UNCERTAINTY_MEASURE_WITH_UNIT(LENGTH_MEASURE(0.01),#74524,
'DISTANCE_ACCURACY_VALUE',
'Maximum model space distance between geometric entities at asserted c
onnectivities');
#74512=UNCERTAINTY_MEASURE_WITH_UNIT(LENGTH_MEASURE(0.01),#74524,
'DISTANCE_ACCURACY_VALUE',
'Maximum model space distance between geometric entities at asserted c
onnectivities');
#74515=(
GEOMETRIC_REPRESENTATION_CONTEXT(3)
GLOBAL_UNCERTAINTY_ASSIGNED_CONTEXT((#74504))
GLOBAL_UNIT_ASSIGNED_CONTEXT((#74524,#74526,#74527))
REPRESENTATION_CONTEXT('','3D')
);
#74523=(
GEOMETRIC_REPRESENTATION_CONTEXT(3)
GLOBAL_UNCERTAINTY_ASSIGNED_CONTEXT((#74512))
GLOBAL_UNIT_ASSIGNED_CONTEXT((#74524,#74526,#74527))
REPRESENTATION_CONTEXT('','3D')
);
#74524=(
LENGTH_UNIT()
NAMED_UNIT(*)
SI_UNIT(.MILLI.,.METRE.)
);
#74526=(
NAMED_UNIT(*)
PLANE_ANGLE_UNIT()
SI_UNIT($,.RADIAN.)
);
#74527=(
NAMED_UNIT(*)
SI_UNIT($,.STERADIAN.)
SOLID_ANGLE_UNIT()
);
#74530=SHAPE_DEFINITION_REPRESENTATION(#74540,#74559);
#74540=PRODUCT_DEFINITION_SHAPE('',$,#74570);
#74559=SHAPE_REPRESENTATION('',(#4883),#74515);
#74567=PRODUCT_DEFINITION_CONTEXT('part definition',#74599,'design');
#74570=PRODUCT_DEFINITION('Clamp_03','Clamp_03',#74580,#74567);
#74580=PRODUCT_DEFINITION_FORMATION('',$,#74603);
#74599=APPLICATION_CONTEXT(
'Core Data for Automotive Mechanical Design Process');
#74600=PRODUCT_CONTEXT('part definition',#74599,'mechanical');
#74603=PRODUCT('Clamp_03','Clamp_03',$,(#74600));
#74612=PRESENTATION_STYLE_ASSIGNMENT((#74615));
#74615=SURFACE_STYLE_USAGE(.BOTH.,#74618);
#74618=SURFACE_SIDE_STYLE('',(#74621));
#74621=SURFACE_STYLE_FILL_AREA(#74624);
#74624=FILL_AREA_STYLE('Opaque(215,0,0)',(#74627));
#74627=FILL_AREA_STYLE_COLOUR('Opaque(215,0,0)',#74630);
#74630=COLOUR_RGB('Opaque(215,0,0)', 0.09019608, 0.27058824, 0.51372549);
ENDSEC;
END-ISO-10303-21;
